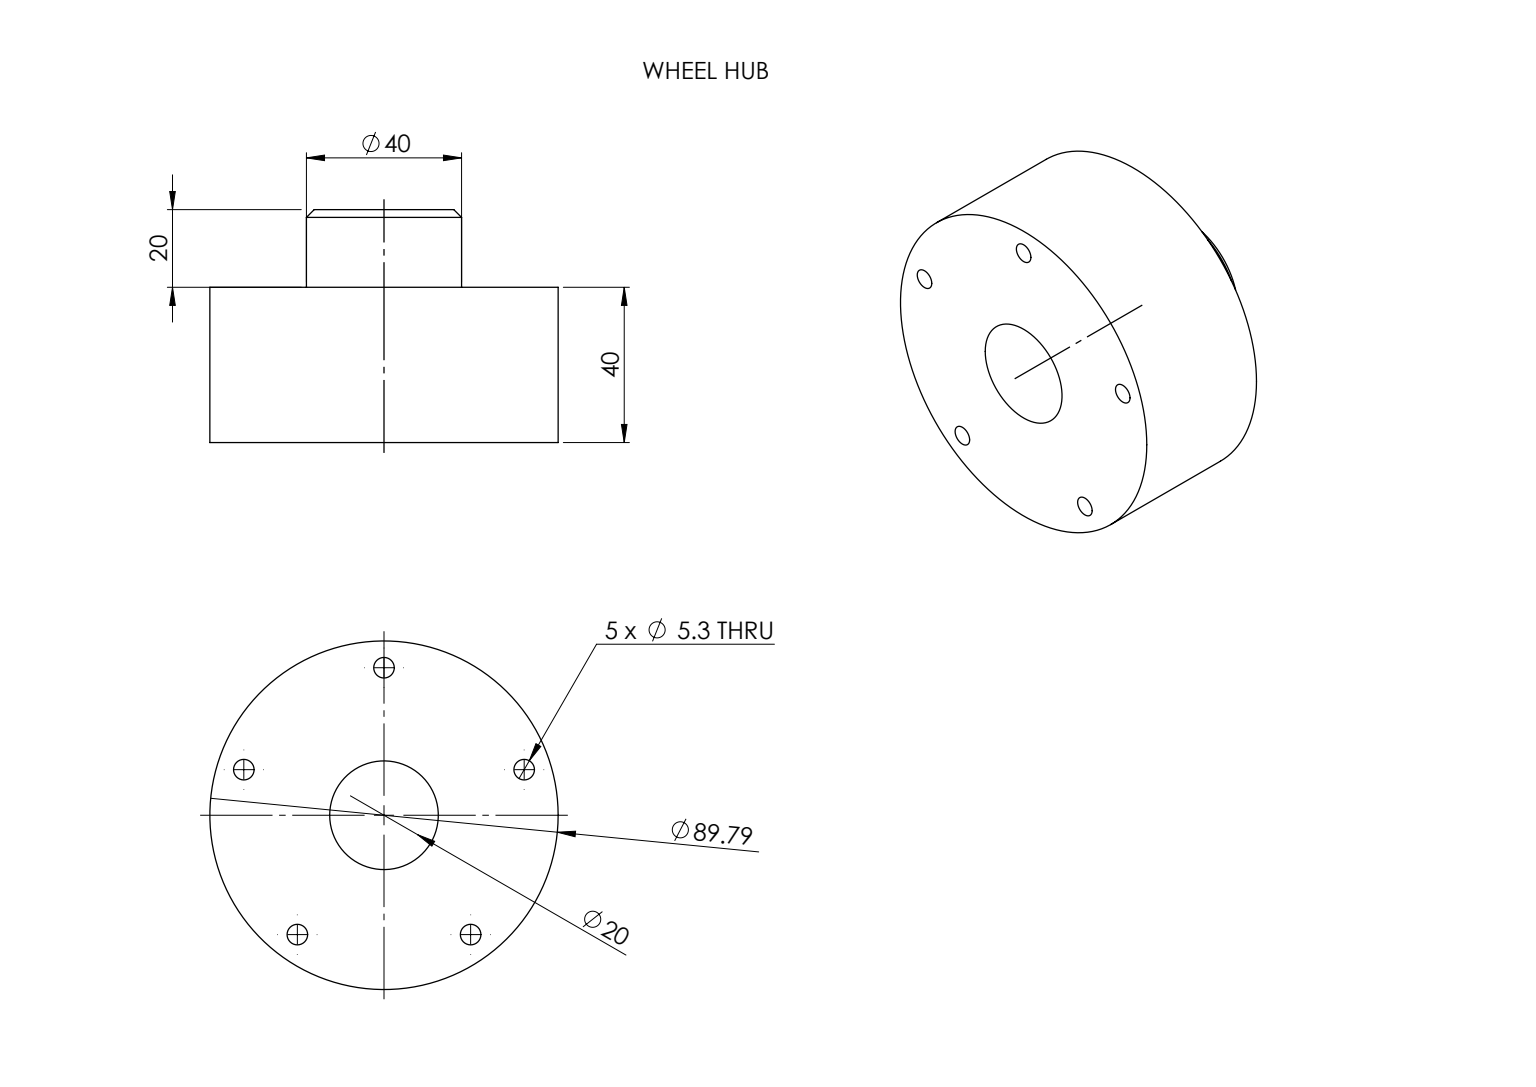
ISO-10303-21;
HEADER;
FILE_DESCRIPTION (('STEP AP214'),
    '1' );
FILE_NAME ('wheel hub.step',
    '2026-10-02T06:35:35',
    ( '' ),
    ( '' ),
    'SwSTEP 2.0',
    'SolidWorks 2026',
    '' );
FILE_SCHEMA (( 'AUTOMOTIVE_DESIGN' ));
ENDSEC;

DATA;
#28=CARTESIAN_POINT ( 'NONE',  ( 0.000000000000000000, 0.000000000000000000, -43.49999999999998579 ) ) ;
#49=CARTESIAN_POINT ( 'NONE',  ( 36.14014761921570340, 11.74264578624841171, -25.50000000000000355 ) ) ;
#103=DIRECTION ( 'NONE',  ( -1.000000000000000000, 0.000000000000000000, 0.000000000000000000 ) ) ;
#141=DIRECTION ( 'NONE',  ( -0.000000000000000000, -0.000000000000000000, -1.000000000000000000 ) ) ;
#154=CIRCLE ( 'NONE', #13005, 2.649999999999985700 ) ;
#173=FACE_OUTER_BOUND ( 'NONE', #9202, .T. ) ;
#234=EDGE_LOOP ( 'NONE', ( #1184, #579, #7849, #6661 ) ) ;
#254=EDGE_CURVE ( 'NONE', #13058, #12937, #12889, .T. ) ;
#255=DIRECTION ( 'NONE',  ( 0.000000000000000000, 0.000000000000000000, -1.000000000000000000 ) ) ;
#276=AXIS2_PLACEMENT_3D ( 'NONE', #8832, #3149, #952 ) ;
#289=CIRCLE ( 'NONE', #11702, 2.649999999999985700 ) ;
#296=CARTESIAN_POINT ( 'NONE',  ( 0.000000000000000000, 0.000000000000000000, 0.000000000000000000 ) ) ;
#313=CARTESIAN_POINT ( 'NONE',  ( -2.449293598294708880E-16, 38.00000000000000000, -25.50000000000000355 ) ) ;
#316=ORIENTED_EDGE ( 'NONE', *, *, #9761, .T. ) ;
#332=PLANE ( 'NONE',  #4860 ) ;
#344=EDGE_CURVE ( 'NONE', #7966, #6056, #4085, .T. ) ;
#357=ORIENTED_EDGE ( 'NONE', *, *, #7968, .F. ) ;
#360=DIRECTION ( 'NONE',  ( -0.000000000000000000, -0.000000000000000000, -1.000000000000000000 ) ) ;
#391=CYLINDRICAL_SURFACE ( 'NONE', #8713, 2.649999999999989253 ) ;
#398=CYLINDRICAL_SURFACE ( 'NONE', #7576, 44.89637028918153305 ) ;
#434=CLOSED_SHELL ( 'NONE', ( #8197, #11127, #13290, #14509, #14180, #5659, #1628, #1611, #1202, #2862, #9335, #12100, #8859, #6336, #14665, #11456, #8232, #5781, #3982, #14557, #1671 ) ) ;
#444=EDGE_CURVE ( 'NONE', #1981, #12602, #7473, .T. ) ;
#455=DIRECTION ( 'NONE',  ( 0.7071067811865444641, 0.000000000000000000, 0.7071067811865505703 ) ) ;
#463=AXIS2_PLACEMENT_3D ( 'NONE', #9565, #3739, #8433 ) ;
#496=FACE_BOUND ( 'NONE', #15028, .T. ) ;
#544=ORIENTED_EDGE ( 'NONE', *, *, #254, .F. ) ;
#551=ORIENTED_EDGE ( 'NONE', *, *, #11963, .T. ) ;
#552=AXIS2_PLACEMENT_3D ( 'NONE', #4395, #14868, #5594 ) ;
#569=DIRECTION ( 'NONE',  ( -1.000000000000000000, 0.000000000000000000, 0.000000000000000000 ) ) ;
#579=ORIENTED_EDGE ( 'NONE', *, *, #13350, .F. ) ;
#584=CIRCLE ( 'NONE', #9055, 2.649999999999985700 ) ;
#604=VERTEX_POINT ( 'NONE', #4820 ) ;
#615=AXIS2_PLACEMENT_3D ( 'NONE', #10778, #2654, #11932 ) ;
#664=VERTEX_POINT ( 'NONE', #8004 ) ;
#679=ORIENTED_EDGE ( 'NONE', *, *, #5242, .T. ) ;
#693=FACE_BOUND ( 'NONE', #8642, .T. ) ;
#722=EDGE_CURVE ( 'NONE', #1196, #1453, #2766, .T. ) ;
#729=PRODUCT_DEFINITION_FORMATION_WITH_SPECIFIED_SOURCE ( 'ANY', '', #6312, .NOT_KNOWN. ) ;
#786=DIRECTION ( 'NONE',  ( 0.000000000000000000, 0.000000000000000000, 1.000000000000000000 ) ) ;
#792=EDGE_CURVE ( 'NONE', #9114, #5585, #14918, .T. ) ;
#796=STYLED_ITEM ( 'NONE', ( #2153 ), #14006 ) ;
#811=ORIENTED_EDGE ( 'NONE', *, *, #3044, .F. ) ;
#812=ORIENTED_EDGE ( 'NONE', *, *, #10110, .F. ) ;
#908=( LENGTH_UNIT ( ) NAMED_UNIT ( * ) SI_UNIT ( .MILLI., .METRE. ) );
#943=DIRECTION ( 'NONE',  ( -0.000000000000000000, -0.000000000000000000, 1.000000000000000000 ) ) ;
#952=DIRECTION ( 'NONE',  ( 1.000000000000000000, 0.000000000000000000, 0.000000000000000000 ) ) ;
#971=( NAMED_UNIT ( * ) SI_UNIT ( $, .STERADIAN. ) SOLID_ANGLE_UNIT ( ) );
#1022=EDGE_CURVE ( 'NONE', #664, #4760, #1315, .T. ) ;
#1039=ORIENTED_EDGE ( 'NONE', *, *, #344, .F. ) ;
#1140=CARTESIAN_POINT ( 'NONE',  ( -44.89637028918153305, 0.000000000000000000, 14.49999999999999822 ) ) ;
#1181=DIRECTION ( 'NONE',  ( 1.000000000000000000, 0.000000000000000000, 0.000000000000000000 ) ) ;
#1184=ORIENTED_EDGE ( 'NONE', *, *, #9617, .F. ) ;
#1191=DIRECTION ( 'NONE',  ( 1.000000000000000000, 0.000000000000000000, 0.000000000000000000 ) ) ;
#1196=VERTEX_POINT ( 'NONE', #5098 ) ;
#1202=ADVANCED_FACE ( 'NONE', ( #14284 ), #398, .T. ) ;
#1204=ORIENTED_EDGE ( 'NONE', *, *, #10110, .T. ) ;
#1232=SHAPE_REPRESENTATION ( 'wheel hub', ( #5108 ), #3871 ) ;
#1234=ORIENTED_EDGE ( 'NONE', *, *, #1022, .T. ) ;
#1293=DIRECTION ( 'NONE',  ( -1.000000000000000000, 0.000000000000000000, 0.000000000000000000 ) ) ;
#1296=CARTESIAN_POINT ( 'NONE',  ( 0.000000000000000000, 0.000000000000000000, 14.49999999999999822 ) ) ;
#1304=CARTESIAN_POINT ( 'NONE',  ( -24.98583958711379083, -30.74264578624812927, -25.50000000000000355 ) ) ;
#1315=LINE ( 'NONE', #8211, #7602 ) ;
#1321=VECTOR ( 'NONE', #14261, 1000.000000000000000 ) ;
#1329=DIRECTION ( 'NONE',  ( -0.000000000000000000, -0.000000000000000000, 1.000000000000000000 ) ) ;
#1386=FACE_OUTER_BOUND ( 'NONE', #1406, .T. ) ;
#1405=DIRECTION ( 'NONE',  ( 0.000000000000000000, 0.000000000000000000, 1.000000000000000000 ) ) ;
#1406=EDGE_LOOP ( 'NONE', ( #12272, #2635, #12944, #14162 ) ) ;
#1436=ORIENTED_EDGE ( 'NONE', *, *, #4515, .F. ) ;
#1443=ORIENTED_EDGE ( 'NONE', *, *, #6310, .F. ) ;
#1446=CARTESIAN_POINT ( 'NONE',  ( -20.00000000000000000, 2.449293598294706513E-15, -25.50000000000000355 ) ) ;
#1453=VERTEX_POINT ( 'NONE', #10254 ) ;
#1546=ORIENTED_EDGE ( 'NONE', *, *, #11963, .F. ) ;
#1551=CARTESIAN_POINT ( 'NONE',  ( -19.68583958711381854, -30.74264578624812927, -25.50000000000000355 ) ) ;
#1555=CARTESIAN_POINT ( 'NONE',  ( 0.000000000000000000, 0.000000000000000000, 14.49999999999999822 ) ) ;
#1608=EDGE_CURVE ( 'NONE', #7966, #10117, #11074, .T. ) ;
#1611=ADVANCED_FACE ( 'NONE', ( #6491 ), #11304, .T. ) ;
#1622=VERTEX_POINT ( 'NONE', #1955 ) ;
#1628=ADVANCED_FACE ( 'NONE', ( #10146 ), #6571, .F. ) ;
#1643=CARTESIAN_POINT ( 'NONE',  ( 36.14014761921570340, 11.74264578624841171, 14.49999999999999822 ) ) ;
#1649=DIRECTION ( 'NONE',  ( -1.000000000000000000, 0.000000000000000000, 0.000000000000000000 ) ) ;
#1671=ADVANCED_FACE ( 'NONE', ( #9378 ), #2394, .F. ) ;
#1676=CARTESIAN_POINT ( 'NONE',  ( -2.649999999999989697, 38.00000000000000000, 14.49999999999999822 ) ) ;
#1682=CARTESIAN_POINT ( 'NONE',  ( 0.000000000000000000, 0.000000000000000000, 14.49999999999999822 ) ) ;
#1690=LINE ( 'NONE', #10643, #5808 ) ;
#1691=DIRECTION ( 'NONE',  ( -0.000000000000000000, -0.000000000000000000, -1.000000000000000000 ) ) ;
#1700=UNCERTAINTY_MEASURE_WITH_UNIT (LENGTH_MEASURE( 1.000000000000000082E-05 ), #4612, 'distance_accuracy_value', 'NONE');
#1710=ORIENTED_EDGE ( 'NONE', *, *, #11180, .F. ) ;
#1717=DIRECTION ( 'NONE',  ( 0.000000000000000000, 0.000000000000000000, 1.000000000000000000 ) ) ;
#1726=EDGE_LOOP ( 'NONE', ( #1204, #13812 ) ) ;
#1730=EDGE_LOOP ( 'NONE', ( #14041, #13678 ) ) ;
#1779=ORIENTED_EDGE ( 'NONE', *, *, #2114, .F. ) ;
#1793=DIRECTION ( 'NONE',  ( -0.000000000000000000, -0.000000000000000000, -1.000000000000000000 ) ) ;
#1806=CARTESIAN_POINT ( 'NONE',  ( -33.49014761921589667, 11.74264578624790190, 14.49999999999999822 ) ) ;
#1824=CARTESIAN_POINT ( 'NONE',  ( 33.49014761921571903, 11.74264578624841171, -25.50000000000000355 ) ) ;
#1832=EDGE_CURVE ( 'NONE', #6056, #10604, #12119, .T. ) ;
#1846=EDGE_CURVE ( 'NONE', #7769, #13374, #8379, .T. ) ;
#1850=ORIENTED_EDGE ( 'NONE', *, *, #10596, .T. ) ;
#1877=CARTESIAN_POINT ( 'NONE',  ( 0.000000000000000000, 0.000000000000000000, -25.50000000000000355 ) ) ;
#1880=ORIENTED_EDGE ( 'NONE', *, *, #4327, .F. ) ;
#1893=AXIS2_PLACEMENT_3D ( 'NONE', #9669, #14480, #14253 ) ;
#1901=ORIENTED_EDGE ( 'NONE', *, *, #12563, .F. ) ;
#1915=FACE_OUTER_BOUND ( 'NONE', #7710, .T. ) ;
#1923=AXIS2_PLACEMENT_3D ( 'NONE', #5073, #9687, #2647 ) ;
#1925=CARTESIAN_POINT ( 'NONE',  ( 2.649999999999988809, 38.00000000000000000, 14.49999999999999822 ) ) ;
#1955=CARTESIAN_POINT ( 'NONE',  ( 18.00000000000000355, 0.000000000000000000, -45.50000000000000000 ) ) ;
#1981=VERTEX_POINT ( 'NONE', #11293 ) ;
#1989=ORIENTED_EDGE ( 'NONE', *, *, #11600, .T. ) ;
#2030=DIRECTION ( 'NONE',  ( 0.000000000000000000, 0.000000000000000000, -1.000000000000000000 ) ) ;
#2086=DIRECTION ( 'NONE',  ( 0.000000000000000000, 0.000000000000000000, 1.000000000000000000 ) ) ;
#2106=DIRECTION ( 'NONE',  ( -1.000000000000000000, 0.000000000000000000, 0.000000000000000000 ) ) ;
#2114=EDGE_CURVE ( 'NONE', #1981, #7885, #154, .T. ) ;
#2128=FACE_BOUND ( 'NONE', #5019, .T. ) ;
#2153=PRESENTATION_STYLE_ASSIGNMENT (( #6769 ) ) ;
#2177=EDGE_LOOP ( 'NONE', ( #8294, #8233 ) ) ;
#2191=EDGE_LOOP ( 'NONE', ( #4825, #12319 ) ) ;
#2204=CARTESIAN_POINT ( 'NONE',  ( -22.33583958711380646, -30.74264578624812927, -25.50000000000000355 ) ) ;
#2209=ORIENTED_EDGE ( 'NONE', *, *, #4162, .T. ) ;
#2214=ADVANCED_BREP_SHAPE_REPRESENTATION ( '', ( #14006, #5108 ), #3871 ) ;
#2241=( GEOMETRIC_REPRESENTATION_CONTEXT ( 3 ) GLOBAL_UNCERTAINTY_ASSIGNED_CONTEXT ( ( #10015 ) ) GLOBAL_UNIT_ASSIGNED_CONTEXT ( ( #7698, #14926, #4667 ) ) REPRESENTATION_CONTEXT ( 'NONE', 'WORKASPACE' ) );
#2250=ORIENTED_EDGE ( 'NONE', *, *, #3584, .T. ) ;
#2269=AXIS2_PLACEMENT_3D ( 'NONE', #6255, #9750, #1649 ) ;
#2276=CIRCLE ( 'NONE', #5174, 20.00000000000000000 ) ;
#2345=LINE ( 'NONE', #8039, #3777 ) ;
#2394=CYLINDRICAL_SURFACE ( 'NONE', #7407, 2.649999999999985700 ) ;
#2405=STYLED_ITEM ( 'NONE', ( #4687 ), #2214 ) ;
#2415=CARTESIAN_POINT ( 'NONE',  ( 36.14014761921570340, 11.74264578624841171, -25.50000000000000355 ) ) ;
#2459=CIRCLE ( 'NONE', #276, 44.89637028918153305 ) ;
#2463=ORIENTED_EDGE ( 'NONE', *, *, #4676, .T. ) ;
#2491=CARTESIAN_POINT ( 'NONE',  ( -22.33583958711380646, -30.74264578624812927, -25.50000000000000355 ) ) ;
#2492=CARTESIAN_POINT ( 'NONE',  ( 44.89637028918153305, 5.498219616798048790E-15, -25.50000000000000355 ) ) ;
#2553=CONICAL_SURFACE ( 'NONE', #13470, 18.00000000000000355, 0.7853981633974439491 ) ;
#2572=CARTESIAN_POINT ( 'NONE',  ( 38.79014761921568777, 11.74264578624841171, -25.50000000000000355 ) ) ;
#2635=ORIENTED_EDGE ( 'NONE', *, *, #3584, .F. ) ;
#2647=DIRECTION ( 'NONE',  ( -1.000000000000000000, 0.000000000000000000, 0.000000000000000000 ) ) ;
#2654=DIRECTION ( 'NONE',  ( 0.000000000000000000, 0.000000000000000000, -1.000000000000000000 ) ) ;
#2674=CYLINDRICAL_SURFACE ( 'NONE', #13644, 2.649999999999985700 ) ;
#2675=CIRCLE ( 'NONE', #4388, 18.00000000000000355 ) ;
#2689=CIRCLE ( 'NONE', #6303, 14.00000000000000000 ) ;
#2708=ORIENTED_EDGE ( 'NONE', *, *, #6734, .F. ) ;
#2727=CIRCLE ( 'NONE', #13165, 2.649999999999985700 ) ;
#2741=DIRECTION ( 'NONE',  ( 0.000000000000000000, 0.000000000000000000, 1.000000000000000000 ) ) ;
#2753=DIRECTION ( 'NONE',  ( 1.000000000000000000, 0.000000000000000000, 0.000000000000000000 ) ) ;
#2764=VERTEX_POINT ( 'NONE', #2970 ) ;
#2766=LINE ( 'NONE', #5196, #7374 ) ;
#2770=CIRCLE ( 'NONE', #11262, 20.00000000000000000 ) ;
#2861=EDGE_CURVE ( 'NONE', #14730, #11825, #5168, .T. ) ;
#2862=ADVANCED_FACE ( 'NONE', ( #8807 ), #5401, .T. ) ;
#2883=DIRECTION ( 'NONE',  ( 1.000000000000000000, 0.000000000000000000, 0.000000000000000000 ) ) ;
#2888=CIRCLE ( 'NONE', #11630, 2.649999999999985700 ) ;
#2911=DIRECTION ( 'NONE',  ( -0.7071067811865444641, 8.659560562354895880E-17, 0.7071067811865505703 ) ) ;
#2926=CARTESIAN_POINT ( 'NONE',  ( -2.449293598294708880E-16, 38.00000000000000000, -25.50000000000000355 ) ) ;
#2939=AXIS2_PLACEMENT_3D ( 'NONE', #10520, #13958, #9300 ) ;
#2954=ORIENTED_EDGE ( 'NONE', *, *, #3044, .T. ) ;
#2970=CARTESIAN_POINT ( 'NONE',  ( 24.98583958711423492, -30.74264578624780597, -25.50000000000000355 ) ) ;
#2993=EDGE_CURVE ( 'NONE', #5519, #12602, #14641, .T. ) ;
#3006=EDGE_LOOP ( 'NONE', ( #12500, #11613, #5941, #2708 ) ) ;
#3033=DIRECTION ( 'NONE',  ( -0.000000000000000000, -0.000000000000000000, -1.000000000000000000 ) ) ;
#3044=EDGE_CURVE ( 'NONE', #2764, #4760, #10509, .T. ) ;
#3054=DIRECTION ( 'NONE',  ( -0.000000000000000000, -0.000000000000000000, -1.000000000000000000 ) ) ;
#3093=EDGE_LOOP ( 'NONE', ( #8891, #811 ) ) ;
#3136=CIRCLE ( 'NONE', #463, 2.649999999999985700 ) ;
#3149=DIRECTION ( 'NONE',  ( 0.000000000000000000, 0.000000000000000000, 1.000000000000000000 ) ) ;
#3265=CARTESIAN_POINT ( 'NONE',  ( 20.00000000000000000, 0.000000000000000000, -43.49999999999998579 ) ) ;
#3286=FACE_OUTER_BOUND ( 'NONE', #11438, .T. ) ;
#3290=CARTESIAN_POINT ( 'NONE',  ( -44.89637028918153305, 0.000000000000000000, -25.50000000000000355 ) ) ;
#3343=FACE_OUTER_BOUND ( 'NONE', #2177, .T. ) ;
#3358=CARTESIAN_POINT ( 'NONE',  ( 0.000000000000000000, 0.000000000000000000, -45.50000000000000000 ) ) ;
#3423=AXIS2_PLACEMENT_3D ( 'NONE', #3994, #10968, #569 ) ;
#3454=DIRECTION ( 'NONE',  ( -1.000000000000000000, 0.000000000000000000, 0.000000000000000000 ) ) ;
#3484=ORIENTED_EDGE ( 'NONE', *, *, #11180, .T. ) ;
#3493=CIRCLE ( 'NONE', #14885, 2.649999999999987477 ) ;
#3511=DIRECTION ( 'NONE',  ( -0.000000000000000000, -0.000000000000000000, -1.000000000000000000 ) ) ;
#3547=AXIS2_PLACEMENT_3D ( 'NONE', #8936, #13571, #12674 ) ;
#3584=EDGE_CURVE ( 'NONE', #604, #11699, #8061, .T. ) ;
#3670=DIRECTION ( 'NONE',  ( -0.000000000000000000, -0.000000000000000000, -1.000000000000000000 ) ) ;
#3688=DIRECTION ( 'NONE',  ( 0.000000000000000000, 0.000000000000000000, -1.000000000000000000 ) ) ;
#3693=ORIENTED_EDGE ( 'NONE', *, *, #10596, .F. ) ;
#3722=AXIS2_PLACEMENT_3D ( 'NONE', #15014, #7091, #1191 ) ;
#3728=AXIS2_PLACEMENT_3D ( 'NONE', #13448, #7669, #12314 ) ;
#3739=DIRECTION ( 'NONE',  ( -0.000000000000000000, -0.000000000000000000, -1.000000000000000000 ) ) ;
#3746=DIRECTION ( 'NONE',  ( -1.000000000000000000, 0.000000000000000000, 0.000000000000000000 ) ) ;
#3748=LINE ( 'NONE', #7370, #9772 ) ;
#3777=VECTOR ( 'NONE', #12681, 1000.000000000000000 ) ;
#3779=FACE_BOUND ( 'NONE', #8908, .T. ) ;
#3783=ORIENTED_EDGE ( 'NONE', *, *, #9761, .F. ) ;
#3787=CARTESIAN_POINT ( 'NONE',  ( -14.00000000000000000, 0.000000000000000000, -45.50000000000000000 ) ) ;
#3850=PRODUCT_DEFINITION ( 'UNKNOWN', '', #729, #11088 ) ;
#3871=( GEOMETRIC_REPRESENTATION_CONTEXT ( 3 ) GLOBAL_UNCERTAINTY_ASSIGNED_CONTEXT ( ( #13249 ) ) GLOBAL_UNIT_ASSIGNED_CONTEXT ( ( #908, #6949, #971 ) ) REPRESENTATION_CONTEXT ( 'NONE', 'WORKASPACE' ) );
#3878=DIRECTION ( 'NONE',  ( -1.000000000000000000, 0.000000000000000000, 0.000000000000000000 ) ) ;
#3905=DIRECTION ( 'NONE',  ( -1.000000000000000000, 0.000000000000000000, 0.000000000000000000 ) ) ;
#3907=DIRECTION ( 'NONE',  ( -1.000000000000000000, 0.000000000000000000, 0.000000000000000000 ) ) ;
#3929=EDGE_LOOP ( 'NONE', ( #14003, #12873, #4799, #14019 ) ) ;
#3977=CARTESIAN_POINT ( 'NONE',  ( 22.33583958711425055, -30.74264578624780597, -25.50000000000000355 ) ) ;
#3982=ADVANCED_FACE ( 'NONE', ( #173 ), #2674, .F. ) ;
#3992=ORIENTED_EDGE ( 'NONE', *, *, #4162, .F. ) ;
#3994=CARTESIAN_POINT ( 'NONE',  ( -36.14014761921588104, 11.74264578624790190, -25.50000000000000355 ) ) ;
#3996=CARTESIAN_POINT ( 'NONE',  ( -38.79014761921587251, 11.74264578624790190, 14.49999999999999822 ) ) ;
#4044=DIRECTION ( 'NONE',  ( -0.000000000000000000, -0.000000000000000000, -1.000000000000000000 ) ) ;
#4066=ORIENTED_EDGE ( 'NONE', *, *, #12665, .F. ) ;
#4078=ORIENTED_EDGE ( 'NONE', *, *, #8401, .T. ) ;
#4085=CIRCLE ( 'NONE', #1893, 2.649999999999989253 ) ;
#4162=EDGE_CURVE ( 'NONE', #5875, #10752, #6907, .T. ) ;
#4173=DIRECTION ( 'NONE',  ( -0.000000000000000000, -0.000000000000000000, -1.000000000000000000 ) ) ;
#4193=FACE_BOUND ( 'NONE', #8365, .T. ) ;
#4196=DIRECTION ( 'NONE',  ( -1.000000000000000000, 0.000000000000000000, 0.000000000000000000 ) ) ;
#4203=ORIENTED_EDGE ( 'NONE', *, *, #1608, .F. ) ;
#4208=DIRECTION ( 'NONE',  ( -0.000000000000000000, -0.000000000000000000, 1.000000000000000000 ) ) ;
#4248=CARTESIAN_POINT ( 'NONE',  ( 0.000000000000000000, 0.000000000000000000, -45.50000000000000000 ) ) ;
#4255=AXIS2_PLACEMENT_3D ( 'NONE', #5276, #2086, #9894 ) ;
#4287=CARTESIAN_POINT ( 'NONE',  ( 20.00000000000000000, 0.000000000000000000, -45.50000000000000000 ) ) ;
#4307=ORIENTED_EDGE ( 'NONE', *, *, #7924, .F. ) ;
#4327=EDGE_CURVE ( 'NONE', #5762, #13414, #11773, .T. ) ;
#4388=AXIS2_PLACEMENT_3D ( 'NONE', #6352, #9557, #3878 ) ;
#4394=CARTESIAN_POINT ( 'NONE',  ( 38.79014761921568777, 11.74264578624841171, -25.50000000000000355 ) ) ;
#4395=CARTESIAN_POINT ( 'NONE',  ( 0.000000000000000000, 0.000000000000000000, 14.49999999999999822 ) ) ;
#4424=ORIENTED_EDGE ( 'NONE', *, *, #2993, .T. ) ;
#4435=DIRECTION ( 'NONE',  ( 1.000000000000000000, 0.000000000000000000, 0.000000000000000000 ) ) ;
#4472=AXIS2_PLACEMENT_3D ( 'NONE', #8660, #8887, #13521 ) ;
#4488=DIRECTION ( 'NONE',  ( 0.000000000000000000, 0.000000000000000000, 1.000000000000000000 ) ) ;
#4503=AXIS2_PLACEMENT_3D ( 'NONE', #5177, #14515, #9791 ) ;
#4512=AXIS2_PLACEMENT_3D ( 'NONE', #1643, #1717, #13263 ) ;
#4515=EDGE_CURVE ( 'NONE', #6851, #13058, #5229, .T. ) ;
#4565=DIRECTION ( 'NONE',  ( 1.000000000000000000, 0.000000000000000000, -0.000000000000000000 ) ) ;
#4575=DIRECTION ( 'NONE',  ( -1.000000000000000000, 0.000000000000000000, 0.000000000000000000 ) ) ;
#4586=VERTEX_POINT ( 'NONE', #13813 ) ;
#4612=( LENGTH_UNIT ( ) NAMED_UNIT ( * ) SI_UNIT ( .MILLI., .METRE. ) );
#4615=AXIS2_PLACEMENT_3D ( 'NONE', #13859, #10426, #3454 ) ;
#4617=DIRECTION ( 'NONE',  ( -0.000000000000000000, -0.000000000000000000, -1.000000000000000000 ) ) ;
#4632=AXIS2_PLACEMENT_3D ( 'NONE', #1296, #7042, #4565 ) ;
#4645=CIRCLE ( 'NONE', #9712, 2.649999999999985700 ) ;
#4667=( NAMED_UNIT ( * ) SI_UNIT ( $, .STERADIAN. ) SOLID_ANGLE_UNIT ( ) );
#4676=EDGE_CURVE ( 'NONE', #11699, #13414, #9535, .T. ) ;
#4687=PRESENTATION_STYLE_ASSIGNMENT (( #14788 ) ) ;
#4760=VERTEX_POINT ( 'NONE', #7103 ) ;
#4784=FACE_OUTER_BOUND ( 'NONE', #11618, .T. ) ;
#4796=CARTESIAN_POINT ( 'NONE',  ( 33.49014761921571903, 11.74264578624841171, 14.49999999999999822 ) ) ;
#4799=ORIENTED_EDGE ( 'NONE', *, *, #11826, .T. ) ;
#4804=VECTOR ( 'NONE', #5750, 1000.000000000000000 ) ;
#4820=CARTESIAN_POINT ( 'NONE',  ( -14.00000000000000000, 0.000000000000000000, 14.49999999999999822 ) ) ;
#4825=ORIENTED_EDGE ( 'NONE', *, *, #7977, .F. ) ;
#4834=DIRECTION ( 'NONE',  ( -0.000000000000000000, -0.000000000000000000, -1.000000000000000000 ) ) ;
#4860=AXIS2_PLACEMENT_3D ( 'NONE', #10728, #6164, #13241 ) ;
#4871=CYLINDRICAL_SURFACE ( 'NONE', #6660, 2.649999999999989253 ) ;
#4970=FACE_BOUND ( 'NONE', #5840, .T. ) ;
#5006=EDGE_LOOP ( 'NONE', ( #6244, #9510, #13738, #4424 ) ) ;
#5019=EDGE_LOOP ( 'NONE', ( #1039, #1546 ) ) ;
#5044=CARTESIAN_POINT ( 'NONE',  ( 0.000000000000000000, 0.000000000000000000, -25.50000000000000355 ) ) ;
#5073=CARTESIAN_POINT ( 'NONE',  ( 0.000000000000000000, 0.000000000000000000, 14.49999999999999822 ) ) ;
#5095=AXIS2_PLACEMENT_3D ( 'NONE', #14277, #7434, #7357 ) ;
#5098=CARTESIAN_POINT ( 'NONE',  ( -18.00000000000000355, 2.326828918379971365E-15, -45.50000000000000000 ) ) ;
#5108=AXIS2_PLACEMENT_3D ( 'NONE', #296, #6125, #10768 ) ;
#5168=CIRCLE ( 'NONE', #6618, 2.649999999999985700 ) ;
#5174=AXIS2_PLACEMENT_3D ( 'NONE', #12943, #1405, #6092 ) ;
#5177=CARTESIAN_POINT ( 'NONE',  ( -36.14014761921588104, 11.74264578624790190, 14.49999999999999822 ) ) ;
#5196=CARTESIAN_POINT ( 'NONE',  ( -18.00000000000000355, 2.204364238465235822E-15, -45.50000000000000000 ) ) ;
#5205=LINE ( 'NONE', #8259, #10473 ) ;
#5229=CIRCLE ( 'NONE', #3547, 44.89637028918153305 ) ;
#5236=APPLICATION_CONTEXT ( 'automotive_design' ) ;
#5242=EDGE_CURVE ( 'NONE', #7769, #14730, #3748, .T. ) ;
#5276=CARTESIAN_POINT ( 'NONE',  ( 0.000000000000000000, 0.000000000000000000, -25.50000000000000355 ) ) ;
#5296=CARTESIAN_POINT ( 'NONE',  ( -2.649999999999989697, 38.00000000000000000, -25.50000000000000355 ) ) ;
#5324=ORIENTED_EDGE ( 'NONE', *, *, #11600, .F. ) ;
#5333=CIRCLE ( 'NONE', #4615, 2.649999999999985700 ) ;
#5334=CARTESIAN_POINT ( 'NONE',  ( -38.79014761921587251, 11.74264578624790190, -25.50000000000000355 ) ) ;
#5338=CYLINDRICAL_SURFACE ( 'NONE', #13383, 20.00000000000000000 ) ;
#5348=ORIENTED_EDGE ( 'NONE', *, *, #14320, .T. ) ;
#5367=EDGE_CURVE ( 'NONE', #12937, #11617, #11006, .T. ) ;
#5386=CARTESIAN_POINT ( 'NONE',  ( 44.89637028918153305, 5.498219616798048790E-15, 14.49999999999999822 ) ) ;
#5401=CYLINDRICAL_SURFACE ( 'NONE', #3728, 44.89637028918153305 ) ;
#5481=EDGE_LOOP ( 'NONE', ( #1436, #10869, #10187, #544 ) ) ;
#5519=VERTEX_POINT ( 'NONE', #8425 ) ;
#5526=DIRECTION ( 'NONE',  ( 1.000000000000000000, 0.000000000000000000, 0.000000000000000000 ) ) ;
#5562=EDGE_LOOP ( 'NONE', ( #9322, #316, #679, #9636 ) ) ;
#5580=CARTESIAN_POINT ( 'NONE',  ( -22.33583958711380646, -30.74264578624812927, 14.49999999999999822 ) ) ;
#5585=VERTEX_POINT ( 'NONE', #1446 ) ;
#5594=DIRECTION ( 'NONE',  ( -1.000000000000000000, 0.000000000000000000, 0.000000000000000000 ) ) ;
#5649=DIRECTION ( 'NONE',  ( 0.000000000000000000, 0.000000000000000000, 1.000000000000000000 ) ) ;
#5659=ADVANCED_FACE ( 'NONE', ( #6802 ), #11754, .T. ) ;
#5676=CARTESIAN_POINT ( 'NONE',  ( 0.000000000000000000, 0.000000000000000000, -45.50000000000000000 ) ) ;
#5744=DIRECTION ( 'NONE',  ( -0.000000000000000000, -0.000000000000000000, -1.000000000000000000 ) ) ;
#5750=DIRECTION ( 'NONE',  ( -0.000000000000000000, -0.000000000000000000, -1.000000000000000000 ) ) ;
#5762=VERTEX_POINT ( 'NONE', #3787 ) ;
#5781=ADVANCED_FACE ( 'NONE', ( #14318 ), #12057, .F. ) ;
#5805=SHAPE_REPRESENTATION_RELATIONSHIP ( 'NONE' , 'NONE' ,  #1232, #2214 ) ;
#5808=VECTOR ( 'NONE', #7448, 1000.000000000000000 ) ;
#5809=CARTESIAN_POINT ( 'NONE',  ( -2.449293598294708880E-16, 38.00000000000000000, -25.50000000000000355 ) ) ;
#5840=EDGE_LOOP ( 'NONE', ( #1880, #3693 ) ) ;
#5875=VERTEX_POINT ( 'NONE', #3996 ) ;
#5922=DIRECTION ( 'NONE',  ( -0.000000000000000000, -0.000000000000000000, -1.000000000000000000 ) ) ;
#5941=ORIENTED_EDGE ( 'NONE', *, *, #6210, .F. ) ;
#5957=CARTESIAN_POINT ( 'NONE',  ( 0.000000000000000000, 0.000000000000000000, -25.50000000000000355 ) ) ;
#5980=CARTESIAN_POINT ( 'NONE',  ( 22.33583958711425055, -30.74264578624780597, 14.49999999999999822 ) ) ;
#5982=ORIENTED_EDGE ( 'NONE', *, *, #7977, .T. ) ;
#6012=EDGE_CURVE ( 'NONE', #11617, #12937, #8599, .T. ) ;
#6025=FACE_BOUND ( 'NONE', #3093, .T. ) ;
#6045=LINE ( 'NONE', #2572, #1321 ) ;
#6056=VERTEX_POINT ( 'NONE', #1925 ) ;
#6085=APPLICATION_CONTEXT ( 'automotive_design' ) ;
#6092=DIRECTION ( 'NONE',  ( -1.000000000000000000, 0.000000000000000000, 0.000000000000000000 ) ) ;
#6101=ORIENTED_EDGE ( 'NONE', *, *, #6734, .T. ) ;
#6117=CARTESIAN_POINT ( 'NONE',  ( -19.68583958711381854, -30.74264578624812927, -25.50000000000000355 ) ) ;
#6125=DIRECTION ( 'NONE',  ( 0.000000000000000000, 0.000000000000000000, 1.000000000000000000 ) ) ;
#6158=EDGE_LOOP ( 'NONE', ( #8298, #9643, #7961, #4203 ) ) ;
#6164=DIRECTION ( 'NONE',  ( 0.000000000000000000, 0.000000000000000000, -1.000000000000000000 ) ) ;
#6167=CARTESIAN_POINT ( 'NONE',  ( -20.00000000000000000, 2.449293598294706513E-15, -45.50000000000000000 ) ) ;
#6174=VECTOR ( 'NONE', #6977, 1000.000000000000000 ) ;
#6201=CARTESIAN_POINT ( 'NONE',  ( 14.00000000000000000, 1.714505518806294638E-15, 14.49999999999999822 ) ) ;
#6210=EDGE_CURVE ( 'NONE', #11466, #1453, #11158, .T. ) ;
#6215=LINE ( 'NONE', #14276, #9954 ) ;
#6230=EDGE_CURVE ( 'NONE', #4760, #2764, #5333, .T. ) ;
#6244=ORIENTED_EDGE ( 'NONE', *, *, #444, .F. ) ;
#6252=ORIENTED_EDGE ( 'NONE', *, *, #7073, .T. ) ;
#6255=CARTESIAN_POINT ( 'NONE',  ( 22.33583958711425055, -30.74264578624780597, -25.50000000000000355 ) ) ;
#6303=AXIS2_PLACEMENT_3D ( 'NONE', #11839, #8553, #11919 ) ;
#6310=EDGE_CURVE ( 'NONE', #604, #5762, #1690, .T. ) ;
#6312=PRODUCT ( 'wheel hub', 'wheel hub', '', ( #9272 ) ) ;
#6316=CIRCLE ( 'NONE', #7047, 2.649999999999987477 ) ;
#6336=ADVANCED_FACE ( 'NONE', ( #8590, #4970 ), #332, .T. ) ;
#6352=CARTESIAN_POINT ( 'NONE',  ( 0.000000000000000000, 0.000000000000000000, -45.50000000000000000 ) ) ;
#6398=ORIENTED_EDGE ( 'NONE', *, *, #8604, .F. ) ;
#6401=DIRECTION ( 'NONE',  ( -1.000000000000000000, 0.000000000000000000, 0.000000000000000000 ) ) ;
#6441=EDGE_LOOP ( 'NONE', ( #13074, #11099 ) ) ;
#6491=FACE_OUTER_BOUND ( 'NONE', #3929, .T. ) ;
#6506=FACE_OUTER_BOUND ( 'NONE', #9509, .T. ) ;
#6571=CYLINDRICAL_SURFACE ( 'NONE', #552, 14.00000000000000000 ) ;
#6618=AXIS2_PLACEMENT_3D ( 'NONE', #14596, #3054, #4196 ) ;
#6623=CIRCLE ( 'NONE', #12454, 18.00000000000000355 ) ;
#6660=AXIS2_PLACEMENT_3D ( 'NONE', #9188, #5922, #8357 ) ;
#6661=ORIENTED_EDGE ( 'NONE', *, *, #5367, .T. ) ;
#6667=DIRECTION ( 'NONE',  ( 1.000000000000000000, 0.000000000000000000, 0.000000000000000000 ) ) ;
#6716=ORIENTED_EDGE ( 'NONE', *, *, #8401, .F. ) ;
#6734=EDGE_CURVE ( 'NONE', #1622, #11466, #6215, .T. ) ;
#6737=DIRECTION ( 'NONE',  ( -0.000000000000000000, -0.000000000000000000, -1.000000000000000000 ) ) ;
#6769=SURFACE_STYLE_USAGE ( .BOTH. , #7925 ) ;
#6793=SURFACE_STYLE_FILL_AREA ( #12740 ) ;
#6802=FACE_OUTER_BOUND ( 'NONE', #3006, .T. ) ;
#6816=CARTESIAN_POINT ( 'NONE',  ( 22.33583958711425055, -30.74264578624780597, -25.50000000000000355 ) ) ;
#6820=DIRECTION ( 'NONE',  ( -0.000000000000000000, -0.000000000000000000, -1.000000000000000000 ) ) ;
#6851=VERTEX_POINT ( 'NONE', #8018 ) ;
#6877=DIRECTION ( 'NONE',  ( -1.000000000000000000, 0.000000000000000000, 0.000000000000000000 ) ) ;
#6896=CYLINDRICAL_SURFACE ( 'NONE', #13564, 2.649999999999985700 ) ;
#6907=CIRCLE ( 'NONE', #4503, 2.649999999999985700 ) ;
#6949=( NAMED_UNIT ( * ) PLANE_ANGLE_UNIT ( ) SI_UNIT ( $, .RADIAN. ) );
#6977=DIRECTION ( 'NONE',  ( -0.000000000000000000, -0.000000000000000000, -1.000000000000000000 ) ) ;
#7015=AXIS2_PLACEMENT_3D ( 'NONE', #28, #5649, #103 ) ;
#7042=DIRECTION ( 'NONE',  ( 0.000000000000000000, 0.000000000000000000, 1.000000000000000000 ) ) ;
#7047=AXIS2_PLACEMENT_3D ( 'NONE', #5809, #12811, #11542 ) ;
#7054=CYLINDRICAL_SURFACE ( 'NONE', #10657, 2.649999999999985700 ) ;
#7073=EDGE_CURVE ( 'NONE', #10743, #7688, #7293, .T. ) ;
#7083=ORIENTED_EDGE ( 'NONE', *, *, #444, .T. ) ;
#7091=DIRECTION ( 'NONE',  ( 0.000000000000000000, 0.000000000000000000, 1.000000000000000000 ) ) ;
#7103=CARTESIAN_POINT ( 'NONE',  ( 19.68583958711426263, -30.74264578624780597, -25.50000000000000355 ) ) ;
#7153=VECTOR ( 'NONE', #7321, 1000.000000000000000 ) ;
#7172=CARTESIAN_POINT ( 'NONE',  ( 2.649999999999988809, 38.00000000000000000, -25.50000000000000355 ) ) ;
#7207=FACE_OUTER_BOUND ( 'NONE', #12076, .T. ) ;
#7216=DIRECTION ( 'NONE',  ( -1.000000000000000000, 0.000000000000000000, 0.000000000000000000 ) ) ;
#7232=CIRCLE ( 'NONE', #10403, 2.649999999999985700 ) ;
#7293=CIRCLE ( 'NONE', #2939, 2.649999999999985700 ) ;
#7300=CYLINDRICAL_SURFACE ( 'NONE', #10970, 2.649999999999985700 ) ;
#7307=COLOUR_RGB ( '', 0.08235294, 0.09019608, 0.10196078) ;
#7320=DIRECTION ( 'NONE',  ( 1.000000000000000000, 0.000000000000000000, -0.000000000000000000 ) ) ;
#7321=DIRECTION ( 'NONE',  ( -0.000000000000000000, -0.000000000000000000, -1.000000000000000000 ) ) ;
#7327=CARTESIAN_POINT ( 'NONE',  ( -22.33583958711380646, -30.74264578624812927, -25.50000000000000355 ) ) ;
#7357=DIRECTION ( 'NONE',  ( -1.000000000000000000, 0.000000000000000000, 0.000000000000000000 ) ) ;
#7370=CARTESIAN_POINT ( 'NONE',  ( 33.49014761921571903, 11.74264578624841171, -25.50000000000000355 ) ) ;
#7372=VECTOR ( 'NONE', #360, 1000.000000000000000 ) ;
#7374=VECTOR ( 'NONE', #2911, 1000.000000000000000 ) ;
#7379=FACE_OUTER_BOUND ( 'NONE', #11819, .T. ) ;
#7407=AXIS2_PLACEMENT_3D ( 'NONE', #49, #5744, #8021 ) ;
#7434=DIRECTION ( 'NONE',  ( -0.000000000000000000, -0.000000000000000000, -1.000000000000000000 ) ) ;
#7448=DIRECTION ( 'NONE',  ( -0.000000000000000000, -0.000000000000000000, -1.000000000000000000 ) ) ;
#7473=LINE ( 'NONE', #6117, #7372 ) ;
#7478=ORIENTED_EDGE ( 'NONE', *, *, #14359, .T. ) ;
#7533=PRODUCT_DEFINITION_SHAPE ( 'NONE', 'NONE',  #3850 ) ;
#7576=AXIS2_PLACEMENT_3D ( 'NONE', #1682, #4044, #3746 ) ;
#7596=ORIENTED_EDGE ( 'NONE', *, *, #11684, .T. ) ;
#7602=VECTOR ( 'NONE', #12927, 1000.000000000000000 ) ;
#7629=AXIS2_PLACEMENT_3D ( 'NONE', #7327, #4834, #14398 ) ;
#7659=ORIENTED_EDGE ( 'NONE', *, *, #14359, .F. ) ;
#7669=DIRECTION ( 'NONE',  ( -0.000000000000000000, -0.000000000000000000, -1.000000000000000000 ) ) ;
#7688=VERTEX_POINT ( 'NONE', #5334 ) ;
#7698=( LENGTH_UNIT ( ) NAMED_UNIT ( * ) SI_UNIT ( .MILLI., .METRE. ) );
#7710=EDGE_LOOP ( 'NONE', ( #4066, #10920, #5348, #8639 ) ) ;
#7750=DIRECTION ( 'NONE',  ( 1.000000000000000000, 0.000000000000000000, 0.000000000000000000 ) ) ;
#7769=VERTEX_POINT ( 'NONE', #4796 ) ;
#7820=CIRCLE ( 'NONE', #3722, 2.649999999999989253 ) ;
#7849=ORIENTED_EDGE ( 'NONE', *, *, #254, .T. ) ;
#7885=VERTEX_POINT ( 'NONE', #12084 ) ;
#7924=EDGE_CURVE ( 'NONE', #7885, #1981, #7232, .T. ) ;
#7925=SURFACE_SIDE_STYLE ('',( #12274 ) ) ;
#7959=FACE_OUTER_BOUND ( 'NONE', #9307, .T. ) ;
#7961=ORIENTED_EDGE ( 'NONE', *, *, #12347, .T. ) ;
#7966=VERTEX_POINT ( 'NONE', #1676 ) ;
#7968=EDGE_CURVE ( 'NONE', #11825, #14730, #3136, .T. ) ;
#7977=EDGE_CURVE ( 'NONE', #664, #4586, #2888, .T. ) ;
#8004=CARTESIAN_POINT ( 'NONE',  ( 19.68583958711426263, -30.74264578624780597, 14.49999999999999822 ) ) ;
#8018=CARTESIAN_POINT ( 'NONE',  ( 44.89637028918153305, 5.498219616798048790E-15, 14.49999999999999822 ) ) ;
#8021=DIRECTION ( 'NONE',  ( -1.000000000000000000, 0.000000000000000000, 0.000000000000000000 ) ) ;
#8039=CARTESIAN_POINT ( 'NONE',  ( -33.49014761921589667, 11.74264578624790190, -25.50000000000000355 ) ) ;
#8042=CYLINDRICAL_SURFACE ( 'NONE', #9193, 2.649999999999985700 ) ;
#8061=CIRCLE ( 'NONE', #9998, 14.00000000000000000 ) ;
#8197=ADVANCED_FACE ( 'NONE', ( #4784 ), #8042, .F. ) ;
#8202=CARTESIAN_POINT ( 'NONE',  ( 24.98583958711423492, -30.74264578624780597, -25.50000000000000355 ) ) ;
#8211=CARTESIAN_POINT ( 'NONE',  ( 19.68583958711426263, -30.74264578624780597, -25.50000000000000355 ) ) ;
#8232=ADVANCED_FACE ( 'NONE', ( #7959 ), #6896, .F. ) ;
#8233=ORIENTED_EDGE ( 'NONE', *, *, #4515, .T. ) ;
#8259=CARTESIAN_POINT ( 'NONE',  ( -38.79014761921587251, 11.74264578624790190, -25.50000000000000355 ) ) ;
#8294=ORIENTED_EDGE ( 'NONE', *, *, #13350, .T. ) ;
#8298=ORIENTED_EDGE ( 'NONE', *, *, #344, .T. ) ;
#8357=DIRECTION ( 'NONE',  ( -1.000000000000000000, 0.000000000000000000, 0.000000000000000000 ) ) ;
#8362=CARTESIAN_POINT ( 'NONE',  ( 22.33583958711425055, -30.74264578624780597, 14.49999999999999822 ) ) ;
#8364=CARTESIAN_POINT ( 'NONE',  ( 20.00000000000000000, 0.000000000000000000, -25.50000000000000355 ) ) ;
#8365=EDGE_LOOP ( 'NONE', ( #2250, #4078 ) ) ;
#8379=CIRCLE ( 'NONE', #4512, 2.649999999999985700 ) ;
#8397=FACE_BOUND ( 'NONE', #1730, .T. ) ;
#8401=EDGE_CURVE ( 'NONE', #11699, #604, #8467, .T. ) ;
#8425=CARTESIAN_POINT ( 'NONE',  ( -24.98583958711379083, -30.74264578624812927, -25.50000000000000355 ) ) ;
#8433=DIRECTION ( 'NONE',  ( -1.000000000000000000, 0.000000000000000000, 0.000000000000000000 ) ) ;
#8442=ORIENTED_EDGE ( 'NONE', *, *, #1608, .T. ) ;
#8461=FACE_BOUND ( 'NONE', #6441, .T. ) ;
#8467=CIRCLE ( 'NONE', #1923, 14.00000000000000000 ) ;
#8501=DIRECTION ( 'NONE',  ( 0.000000000000000000, 0.000000000000000000, 1.000000000000000000 ) ) ;
#8516=ORIENTED_EDGE ( 'NONE', *, *, #7968, .T. ) ;
#8534=CYLINDRICAL_SURFACE ( 'NONE', #3423, 2.649999999999985700 ) ;
#8553=DIRECTION ( 'NONE',  ( 0.000000000000000000, 0.000000000000000000, -1.000000000000000000 ) ) ;
#8571=DIRECTION ( 'NONE',  ( -0.000000000000000000, -0.000000000000000000, -1.000000000000000000 ) ) ;
#8590=FACE_OUTER_BOUND ( 'NONE', #1726, .T. ) ;
#8599=CIRCLE ( 'NONE', #4255, 44.89637028918153305 ) ;
#8604=EDGE_CURVE ( 'NONE', #10117, #10604, #6316, .T. ) ;
#8625=EDGE_CURVE ( 'NONE', #7688, #10743, #4645, .T. ) ;
#8639=ORIENTED_EDGE ( 'NONE', *, *, #792, .T. ) ;
#8642=EDGE_LOOP ( 'NONE', ( #3992, #7659 ) ) ;
#8660=CARTESIAN_POINT ( 'NONE',  ( 0.000000000000000000, 0.000000000000000000, -25.50000000000000355 ) ) ;
#8705=LINE ( 'NONE', #5386, #11407 ) ;
#8713=AXIS2_PLACEMENT_3D ( 'NONE', #313, #8571, #14213 ) ;
#8807=FACE_OUTER_BOUND ( 'NONE', #234, .T. ) ;
#8832=CARTESIAN_POINT ( 'NONE',  ( 0.000000000000000000, 0.000000000000000000, 14.49999999999999822 ) ) ;
#8836=ORIENTED_EDGE ( 'NONE', *, *, #12347, .F. ) ;
#8859=ADVANCED_FACE ( 'NONE', ( #1915 ), #5338, .T. ) ;
#8887=DIRECTION ( 'NONE',  ( 0.000000000000000000, 0.000000000000000000, 1.000000000000000000 ) ) ;
#8891=ORIENTED_EDGE ( 'NONE', *, *, #6230, .F. ) ;
#8908=EDGE_LOOP ( 'NONE', ( #9874, #14044 ) ) ;
#8936=CARTESIAN_POINT ( 'NONE',  ( 0.000000000000000000, 0.000000000000000000, 14.49999999999999822 ) ) ;
#8950=DIRECTION ( 'NONE',  ( -1.000000000000000000, 0.000000000000000000, 0.000000000000000000 ) ) ;
#8959=AXIS2_PLACEMENT_3D ( 'NONE', #9577, #10726, #2753 ) ;
#9034=AXIS2_PLACEMENT_3D ( 'NONE', #5957, #14312, #7320 ) ;
#9055=AXIS2_PLACEMENT_3D ( 'NONE', #5980, #12904, #11774 ) ;
#9114=VERTEX_POINT ( 'NONE', #8364 ) ;
#9129=ORIENTED_EDGE ( 'NONE', *, *, #13875, .F. ) ;
#9148=DIRECTION ( 'NONE',  ( 0.000000000000000000, 0.000000000000000000, 1.000000000000000000 ) ) ;
#9157=( NAMED_UNIT ( * ) PLANE_ANGLE_UNIT ( ) SI_UNIT ( $, .RADIAN. ) );
#9177=ORIENTED_EDGE ( 'NONE', *, *, #1846, .T. ) ;
#9188=CARTESIAN_POINT ( 'NONE',  ( -2.449293598294708880E-16, 38.00000000000000000, -25.50000000000000355 ) ) ;
#9193=AXIS2_PLACEMENT_3D ( 'NONE', #2415, #6737, #1293 ) ;
#9200=CIRCLE ( 'NONE', #8959, 2.649999999999985700 ) ;
#9202=EDGE_LOOP ( 'NONE', ( #5324, #7478, #9618, #12990 ) ) ;
#9239=DIRECTION ( 'NONE',  ( 1.000000000000000000, 0.000000000000000000, 0.000000000000000000 ) ) ;
#9256=PLANE ( 'NONE',  #4632 ) ;
#9268=LINE ( 'NONE', #8202, #12737 ) ;
#9272=PRODUCT_CONTEXT ( 'NONE', #6085, 'mechanical' ) ;
#9300=DIRECTION ( 'NONE',  ( -1.000000000000000000, 0.000000000000000000, 0.000000000000000000 ) ) ;
#9307=EDGE_LOOP ( 'NONE', ( #1710, #12322, #1234, #12991 ) ) ;
#9322=ORIENTED_EDGE ( 'NONE', *, *, #11684, .F. ) ;
#9324=DIRECTION ( 'NONE',  ( -0.000000000000000000, -0.000000000000000000, -1.000000000000000000 ) ) ;
#9335=ADVANCED_FACE ( 'NONE', ( #12538, #2128, #693, #9942, #14593, #4193, #3343 ), #9256, .T. ) ;
#9378=FACE_OUTER_BOUND ( 'NONE', #5562, .T. ) ;
#9509=EDGE_LOOP ( 'NONE', ( #10769, #812, #6101, #1901 ) ) ;
#9510=ORIENTED_EDGE ( 'NONE', *, *, #2114, .T. ) ;
#9535=LINE ( 'NONE', #11615, #14452 ) ;
#9557=DIRECTION ( 'NONE',  ( 0.000000000000000000, 0.000000000000000000, -1.000000000000000000 ) ) ;
#9565=CARTESIAN_POINT ( 'NONE',  ( 36.14014761921570340, 11.74264578624841171, -25.50000000000000355 ) ) ;
#9577=CARTESIAN_POINT ( 'NONE',  ( 36.14014761921570340, 11.74264578624841171, 14.49999999999999822 ) ) ;
#9617=EDGE_CURVE ( 'NONE', #6851, #11617, #8705, .T. ) ;
#9618=ORIENTED_EDGE ( 'NONE', *, *, #13875, .T. ) ;
#9636=ORIENTED_EDGE ( 'NONE', *, *, #2861, .T. ) ;
#9643=ORIENTED_EDGE ( 'NONE', *, *, #1832, .T. ) ;
#9662=PLANE ( 'NONE',  #9034 ) ;
#9669=CARTESIAN_POINT ( 'NONE',  ( -2.449293598294708880E-16, 38.00000000000000000, 14.49999999999999822 ) ) ;
#9673=ORIENTED_EDGE ( 'NONE', *, *, #6012, .F. ) ;
#9686=CARTESIAN_POINT ( 'NONE',  ( -44.89637028918153305, 0.000000000000000000, 14.49999999999999822 ) ) ;
#9687=DIRECTION ( 'NONE',  ( 0.000000000000000000, 0.000000000000000000, -1.000000000000000000 ) ) ;
#9688=EDGE_LOOP ( 'NONE', ( #11521, #3783 ) ) ;
#9712=AXIS2_PLACEMENT_3D ( 'NONE', #14870, #4617, #6877 ) ;
#9714=CARTESIAN_POINT ( 'NONE',  ( -36.14014761921588104, 11.74264578624790190, -25.50000000000000355 ) ) ;
#9717=DIRECTION ( 'NONE',  ( -0.000000000000000000, -0.000000000000000000, -1.000000000000000000 ) ) ;
#9750=DIRECTION ( 'NONE',  ( -0.000000000000000000, -0.000000000000000000, -1.000000000000000000 ) ) ;
#9761=EDGE_CURVE ( 'NONE', #13374, #7769, #9200, .T. ) ;
#9772=VECTOR ( 'NONE', #9717, 1000.000000000000000 ) ;
#9791=DIRECTION ( 'NONE',  ( 1.000000000000000000, 0.000000000000000000, 0.000000000000000000 ) ) ;
#9874=ORIENTED_EDGE ( 'NONE', *, *, #8625, .F. ) ;
#9894=DIRECTION ( 'NONE',  ( 1.000000000000000000, 0.000000000000000000, 0.000000000000000000 ) ) ;
#9895=FILL_AREA_STYLE ('',( #13477 ) ) ;
#9942=FACE_BOUND ( 'NONE', #10070, .T. ) ;
#9954=VECTOR ( 'NONE', #455, 1000.000000000000000 ) ;
#9959=LINE ( 'NONE', #4287, #10721 ) ;
#9998=AXIS2_PLACEMENT_3D ( 'NONE', #1555, #3688, #11968 ) ;
#10015=UNCERTAINTY_MEASURE_WITH_UNIT (LENGTH_MEASURE( 1.000000000000000082E-05 ), #7698, 'distance_accuracy_value', 'NONE');
#10037=VECTOR ( 'NONE', #1329, 1000.000000000000000 ) ;
#10065=ORIENTED_EDGE ( 'NONE', *, *, #11192, .F. ) ;
#10070=EDGE_LOOP ( 'NONE', ( #4307, #1779 ) ) ;
#10110=EDGE_CURVE ( 'NONE', #1622, #1196, #2675, .T. ) ;
#10117=VERTEX_POINT ( 'NONE', #13142 ) ;
#10146=FACE_OUTER_BOUND ( 'NONE', #10633, .T. ) ;
#10187=ORIENTED_EDGE ( 'NONE', *, *, #6012, .T. ) ;
#10219=ORIENTED_EDGE ( 'NONE', *, *, #5242, .F. ) ;
#10225=FILL_AREA_STYLE_COLOUR ( '', #11142 ) ;
#10254=CARTESIAN_POINT ( 'NONE',  ( -20.00000000000000000, 2.449293598294706513E-15, -43.49999999999998579 ) ) ;
#10403=AXIS2_PLACEMENT_3D ( 'NONE', #14435, #8501, #2883 ) ;
#10409=CARTESIAN_POINT ( 'NONE',  ( -22.33583958711380646, -30.74264578624812927, -25.50000000000000355 ) ) ;
#10426=DIRECTION ( 'NONE',  ( -0.000000000000000000, -0.000000000000000000, -1.000000000000000000 ) ) ;
#10448=SURFACE_SIDE_STYLE ('',( #6793 ) ) ;
#10473=VECTOR ( 'NONE', #9324, 1000.000000000000000 ) ;
#10509=CIRCLE ( 'NONE', #2269, 2.649999999999985700 ) ;
#10520=CARTESIAN_POINT ( 'NONE',  ( -36.14014761921588104, 11.74264578624790190, -25.50000000000000355 ) ) ;
#10596=EDGE_CURVE ( 'NONE', #13414, #5762, #2689, .T. ) ;
#10604=VERTEX_POINT ( 'NONE', #11997 ) ;
#10633=EDGE_LOOP ( 'NONE', ( #6716, #2463, #1850, #1443 ) ) ;
#10643=CARTESIAN_POINT ( 'NONE',  ( -14.00000000000000000, 0.000000000000000000, 14.49999999999999822 ) ) ;
#10657=AXIS2_PLACEMENT_3D ( 'NONE', #10409, #13841, #4575 ) ;
#10721=VECTOR ( 'NONE', #4208, 1000.000000000000000 ) ;
#10726=DIRECTION ( 'NONE',  ( 0.000000000000000000, 0.000000000000000000, 1.000000000000000000 ) ) ;
#10728=CARTESIAN_POINT ( 'NONE',  ( 0.000000000000000000, 0.000000000000000000, -45.50000000000000000 ) ) ;
#10732=CARTESIAN_POINT ( 'NONE',  ( 0.000000000000000000, 0.000000000000000000, -45.50000000000000000 ) ) ;
#10743=VERTEX_POINT ( 'NONE', #11222 ) ;
#10752=VERTEX_POINT ( 'NONE', #1806 ) ;
#10768=DIRECTION ( 'NONE',  ( 1.000000000000000000, 0.000000000000000000, 0.000000000000000000 ) ) ;
#10769=ORIENTED_EDGE ( 'NONE', *, *, #722, .F. ) ;
#10778=CARTESIAN_POINT ( 'NONE',  ( 0.000000000000000000, 0.000000000000000000, -45.50000000000000000 ) ) ;
#10824=FACE_OUTER_BOUND ( 'NONE', #13316, .T. ) ;
#10869=ORIENTED_EDGE ( 'NONE', *, *, #9617, .T. ) ;
#10892=FACE_BOUND ( 'NONE', #11278, .T. ) ;
#10920=ORIENTED_EDGE ( 'NONE', *, *, #12563, .T. ) ;
#10968=DIRECTION ( 'NONE',  ( -0.000000000000000000, -0.000000000000000000, -1.000000000000000000 ) ) ;
#10970=AXIS2_PLACEMENT_3D ( 'NONE', #3977, #1691, #3905 ) ;
#10972=DIRECTION ( 'NONE',  ( -0.000000000000000000, -0.000000000000000000, -1.000000000000000000 ) ) ;
#10978=AXIS2_PLACEMENT_3D ( 'NONE', #4248, #11145, #5526 ) ;
#11006=CIRCLE ( 'NONE', #4472, 44.89637028918153305 ) ;
#11074=LINE ( 'NONE', #5296, #13643 ) ;
#11088=PRODUCT_DEFINITION_CONTEXT ( 'detailed design', #5236, 'design' ) ;
#11099=ORIENTED_EDGE ( 'NONE', *, *, #11826, .F. ) ;
#11127=ADVANCED_FACE ( 'NONE', ( #12837 ), #4871, .F. ) ;
#11142=COLOUR_RGB ( '', 0.08235294, 0.09019608, 0.10196078) ;
#11145=DIRECTION ( 'NONE',  ( -0.000000000000000000, -0.000000000000000000, 1.000000000000000000 ) ) ;
#11158=CIRCLE ( 'NONE', #7015, 20.00000000000000000 ) ;
#11180=EDGE_CURVE ( 'NONE', #4586, #2764, #9268, .T. ) ;
#11187=CARTESIAN_POINT ( 'NONE',  ( -36.14014761921588104, 11.74264578624790190, 14.49999999999999822 ) ) ;
#11192=EDGE_CURVE ( 'NONE', #7885, #5519, #14130, .T. ) ;
#11222=CARTESIAN_POINT ( 'NONE',  ( -33.49014761921589667, 11.74264578624790190, -25.50000000000000355 ) ) ;
#11242=CARTESIAN_POINT ( 'NONE',  ( 0.000000000000000000, 0.000000000000000000, -45.50000000000000000 ) ) ;
#11262=AXIS2_PLACEMENT_3D ( 'NONE', #1877, #2030, #2106 ) ;
#11273=AXIS2_PLACEMENT_3D ( 'NONE', #5676, #13739, #9239 ) ;
#11278=EDGE_LOOP ( 'NONE', ( #12803, #357 ) ) ;
#11293=CARTESIAN_POINT ( 'NONE',  ( -19.68583958711381854, -30.74264578624812927, 14.49999999999999822 ) ) ;
#11304=CYLINDRICAL_SURFACE ( 'NONE', #10978, 20.00000000000000000 ) ;
#11349=CARTESIAN_POINT ( 'NONE',  ( 38.79014761921568777, 11.74264578624841171, 14.49999999999999822 ) ) ;
#11407=VECTOR ( 'NONE', #3033, 1000.000000000000000 ) ;
#11438=EDGE_LOOP ( 'NONE', ( #12527, #7083, #14862, #10065 ) ) ;
#11456=ADVANCED_FACE ( 'NONE', ( #6506 ), #2553, .T. ) ;
#11466=VERTEX_POINT ( 'NONE', #3265 ) ;
#11521=ORIENTED_EDGE ( 'NONE', *, *, #1846, .F. ) ;
#11542=DIRECTION ( 'NONE',  ( -1.000000000000000000, 0.000000000000000000, 0.000000000000000000 ) ) ;
#11600=EDGE_CURVE ( 'NONE', #10752, #10743, #2345, .T. ) ;
#11613=ORIENTED_EDGE ( 'NONE', *, *, #722, .T. ) ;
#11615=CARTESIAN_POINT ( 'NONE',  ( 14.00000000000000000, 1.714505518806294638E-15, 14.49999999999999822 ) ) ;
#11617=VERTEX_POINT ( 'NONE', #2492 ) ;
#11618=EDGE_LOOP ( 'NONE', ( #9177, #7596, #8516, #10219 ) ) ;
#11630=AXIS2_PLACEMENT_3D ( 'NONE', #8362, #2741, #12018 ) ;
#11684=EDGE_CURVE ( 'NONE', #13374, #11825, #6045, .T. ) ;
#11696=DIRECTION ( 'NONE',  ( -1.000000000000000000, 0.000000000000000000, 0.000000000000000000 ) ) ;
#11699=VERTEX_POINT ( 'NONE', #6201 ) ;
#11702=AXIS2_PLACEMENT_3D ( 'NONE', #2491, #10972, #11696 ) ;
#11754=CONICAL_SURFACE ( 'NONE', #11273, 18.00000000000000355, 0.7853981633974439491 ) ;
#11773=CIRCLE ( 'NONE', #615, 14.00000000000000000 ) ;
#11774=DIRECTION ( 'NONE',  ( 1.000000000000000000, 0.000000000000000000, 0.000000000000000000 ) ) ;
#11796=ORIENTED_EDGE ( 'NONE', *, *, #1832, .F. ) ;
#11819=EDGE_LOOP ( 'NONE', ( #5982, #3484, #2954, #12530 ) ) ;
#11825=VERTEX_POINT ( 'NONE', #4394 ) ;
#11826=EDGE_CURVE ( 'NONE', #5585, #9114, #2770, .T. ) ;
#11839=CARTESIAN_POINT ( 'NONE',  ( 0.000000000000000000, 0.000000000000000000, -45.50000000000000000 ) ) ;
#11872=MECHANICAL_DESIGN_GEOMETRIC_PRESENTATION_REPRESENTATION('',(#2405),#15026);
#11919=DIRECTION ( 'NONE',  ( -1.000000000000000000, 0.000000000000000000, 0.000000000000000000 ) ) ;
#11932=DIRECTION ( 'NONE',  ( -1.000000000000000000, 0.000000000000000000, 0.000000000000000000 ) ) ;
#11962=LINE ( 'NONE', #6167, #10037 ) ;
#11963=EDGE_CURVE ( 'NONE', #6056, #7966, #7820, .T. ) ;
#11968=DIRECTION ( 'NONE',  ( -1.000000000000000000, 0.000000000000000000, 0.000000000000000000 ) ) ;
#11997=CARTESIAN_POINT ( 'NONE',  ( 2.649999999999987033, 38.00000000000000000, -25.50000000000000355 ) ) ;
#12018=DIRECTION ( 'NONE',  ( 1.000000000000000000, 0.000000000000000000, 0.000000000000000000 ) ) ;
#12057=CYLINDRICAL_SURFACE ( 'NONE', #7629, 2.649999999999985700 ) ;
#12076=EDGE_LOOP ( 'NONE', ( #11796, #551, #8442, #12642 ) ) ;
#12084=CARTESIAN_POINT ( 'NONE',  ( -24.98583958711379083, -30.74264578624812927, 14.49999999999999822 ) ) ;
#12100=ADVANCED_FACE ( 'NONE', ( #10892, #496, #3779, #8397, #6025, #8461, #10824 ), #9662, .F. ) ;
#12119=LINE ( 'NONE', #7172, #7153 ) ;
#12272=ORIENTED_EDGE ( 'NONE', *, *, #4676, .F. ) ;
#12274=SURFACE_STYLE_FILL_AREA ( #9895 ) ;
#12314=DIRECTION ( 'NONE',  ( -1.000000000000000000, 0.000000000000000000, 0.000000000000000000 ) ) ;
#12319=ORIENTED_EDGE ( 'NONE', *, *, #12870, .F. ) ;
#12322=ORIENTED_EDGE ( 'NONE', *, *, #12870, .T. ) ;
#12347=EDGE_CURVE ( 'NONE', #10604, #10117, #3493, .T. ) ;
#12454=AXIS2_PLACEMENT_3D ( 'NONE', #10732, #255, #3907 ) ;
#12500=ORIENTED_EDGE ( 'NONE', *, *, #12526, .F. ) ;
#12526=EDGE_CURVE ( 'NONE', #1196, #1622, #6623, .T. ) ;
#12527=ORIENTED_EDGE ( 'NONE', *, *, #7924, .T. ) ;
#12530=ORIENTED_EDGE ( 'NONE', *, *, #1022, .F. ) ;
#12538=FACE_BOUND ( 'NONE', #9688, .T. ) ;
#12563=EDGE_CURVE ( 'NONE', #1453, #11466, #2276, .T. ) ;
#12601=DIRECTION ( 'NONE',  ( -0.000000000000000000, -0.000000000000000000, -1.000000000000000000 ) ) ;
#12602=VERTEX_POINT ( 'NONE', #1551 ) ;
#12642=ORIENTED_EDGE ( 'NONE', *, *, #8604, .T. ) ;
#12665=EDGE_CURVE ( 'NONE', #1453, #5585, #11962, .T. ) ;
#12674=DIRECTION ( 'NONE',  ( 1.000000000000000000, 0.000000000000000000, 0.000000000000000000 ) ) ;
#12681=DIRECTION ( 'NONE',  ( -0.000000000000000000, -0.000000000000000000, -1.000000000000000000 ) ) ;
#12737=VECTOR ( 'NONE', #3511, 1000.000000000000000 ) ;
#12740=FILL_AREA_STYLE ('',( #10225 ) ) ;
#12803=ORIENTED_EDGE ( 'NONE', *, *, #2861, .F. ) ;
#12811=DIRECTION ( 'NONE',  ( -0.000000000000000000, -0.000000000000000000, -1.000000000000000000 ) ) ;
#12837=FACE_OUTER_BOUND ( 'NONE', #6158, .T. ) ;
#12870=EDGE_CURVE ( 'NONE', #4586, #664, #584, .T. ) ;
#12873=ORIENTED_EDGE ( 'NONE', *, *, #12665, .T. ) ;
#12889=LINE ( 'NONE', #1140, #4804 ) ;
#12904=DIRECTION ( 'NONE',  ( 0.000000000000000000, 0.000000000000000000, 1.000000000000000000 ) ) ;
#12927=DIRECTION ( 'NONE',  ( -0.000000000000000000, -0.000000000000000000, -1.000000000000000000 ) ) ;
#12931=AXIS2_PLACEMENT_3D ( 'NONE', #2204, #6820, #8950 ) ;
#12937=VERTEX_POINT ( 'NONE', #3290 ) ;
#12943=CARTESIAN_POINT ( 'NONE',  ( 0.000000000000000000, 0.000000000000000000, -43.49999999999998579 ) ) ;
#12944=ORIENTED_EDGE ( 'NONE', *, *, #6310, .T. ) ;
#12972=AXIS2_PLACEMENT_3D ( 'NONE', #5044, #13024, #14236 ) ;
#12990=ORIENTED_EDGE ( 'NONE', *, *, #8625, .T. ) ;
#12991=ORIENTED_EDGE ( 'NONE', *, *, #6230, .T. ) ;
#13005=AXIS2_PLACEMENT_3D ( 'NONE', #5580, #9148, #1181 ) ;
#13024=DIRECTION ( 'NONE',  ( 0.000000000000000000, 0.000000000000000000, -1.000000000000000000 ) ) ;
#13058=VERTEX_POINT ( 'NONE', #9686 ) ;
#13074=ORIENTED_EDGE ( 'NONE', *, *, #792, .F. ) ;
#13142=CARTESIAN_POINT ( 'NONE',  ( -2.649999999999987921, 38.00000000000000000, -25.50000000000000355 ) ) ;
#13146=CYLINDRICAL_SURFACE ( 'NONE', #5095, 14.00000000000000000 ) ;
#13165=AXIS2_PLACEMENT_3D ( 'NONE', #11187, #786, #7750 ) ;
#13241=DIRECTION ( 'NONE',  ( -1.000000000000000000, 0.000000000000000000, -0.000000000000000000 ) ) ;
#13249=UNCERTAINTY_MEASURE_WITH_UNIT (LENGTH_MEASURE( 1.000000000000000082E-05 ), #908, 'distance_accuracy_value', 'NONE');
#13263=DIRECTION ( 'NONE',  ( 1.000000000000000000, 0.000000000000000000, 0.000000000000000000 ) ) ;
#13290=ADVANCED_FACE ( 'NONE', ( #14386 ), #8534, .F. ) ;
#13316=EDGE_LOOP ( 'NONE', ( #14109, #9673 ) ) ;
#13350=EDGE_CURVE ( 'NONE', #13058, #6851, #2459, .T. ) ;
#13374=VERTEX_POINT ( 'NONE', #11349 ) ;
#13383=AXIS2_PLACEMENT_3D ( 'NONE', #3358, #943, #4435 ) ;
#13414=VERTEX_POINT ( 'NONE', #13474 ) ;
#13448=CARTESIAN_POINT ( 'NONE',  ( 0.000000000000000000, 0.000000000000000000, 14.49999999999999822 ) ) ;
#13470=AXIS2_PLACEMENT_3D ( 'NONE', #11242, #4488, #6667 ) ;
#13474=CARTESIAN_POINT ( 'NONE',  ( 14.00000000000000000, 1.714505518806294638E-15, -45.50000000000000000 ) ) ;
#13477=FILL_AREA_STYLE_COLOUR ( '', #7307 ) ;
#13521=DIRECTION ( 'NONE',  ( 1.000000000000000000, 0.000000000000000000, 0.000000000000000000 ) ) ;
#13564=AXIS2_PLACEMENT_3D ( 'NONE', #6816, #12601, #13904 ) ;
#13571=DIRECTION ( 'NONE',  ( 0.000000000000000000, 0.000000000000000000, 1.000000000000000000 ) ) ;
#13639=MECHANICAL_DESIGN_GEOMETRIC_PRESENTATION_REPRESENTATION('',(#796),#2241);
#13643=VECTOR ( 'NONE', #4173, 1000.000000000000000 ) ;
#13644=AXIS2_PLACEMENT_3D ( 'NONE', #9714, #3670, #7216 ) ;
#13648=( NAMED_UNIT ( * ) SI_UNIT ( $, .STERADIAN. ) SOLID_ANGLE_UNIT ( ) );
#13678=ORIENTED_EDGE ( 'NONE', *, *, #13873, .F. ) ;
#13738=ORIENTED_EDGE ( 'NONE', *, *, #11192, .T. ) ;
#13739=DIRECTION ( 'NONE',  ( 0.000000000000000000, 0.000000000000000000, 1.000000000000000000 ) ) ;
#13812=ORIENTED_EDGE ( 'NONE', *, *, #12526, .T. ) ;
#13813=CARTESIAN_POINT ( 'NONE',  ( 24.98583958711423492, -30.74264578624780597, 14.49999999999999822 ) ) ;
#13841=DIRECTION ( 'NONE',  ( -0.000000000000000000, -0.000000000000000000, -1.000000000000000000 ) ) ;
#13859=CARTESIAN_POINT ( 'NONE',  ( 22.33583958711425055, -30.74264578624780597, -25.50000000000000355 ) ) ;
#13873=EDGE_CURVE ( 'NONE', #12602, #5519, #289, .T. ) ;
#13875=EDGE_CURVE ( 'NONE', #5875, #7688, #5205, .T. ) ;
#13897=EDGE_LOOP ( 'NONE', ( #2209, #1989, #6252, #9129 ) ) ;
#13904=DIRECTION ( 'NONE',  ( -1.000000000000000000, 0.000000000000000000, 0.000000000000000000 ) ) ;
#13924=SHAPE_DEFINITION_REPRESENTATION ( #7533, #1232 ) ;
#13958=DIRECTION ( 'NONE',  ( -0.000000000000000000, -0.000000000000000000, -1.000000000000000000 ) ) ;
#14003=ORIENTED_EDGE ( 'NONE', *, *, #6210, .T. ) ;
#14006=MANIFOLD_SOLID_BREP ( 'M5 Clearance Hole1', #434 ) ;
#14019=ORIENTED_EDGE ( 'NONE', *, *, #14320, .F. ) ;
#14041=ORIENTED_EDGE ( 'NONE', *, *, #2993, .F. ) ;
#14044=ORIENTED_EDGE ( 'NONE', *, *, #7073, .F. ) ;
#14109=ORIENTED_EDGE ( 'NONE', *, *, #5367, .F. ) ;
#14130=LINE ( 'NONE', #1304, #6174 ) ;
#14162=ORIENTED_EDGE ( 'NONE', *, *, #4327, .T. ) ;
#14180=ADVANCED_FACE ( 'NONE', ( #7379 ), #7300, .F. ) ;
#14213=DIRECTION ( 'NONE',  ( -1.000000000000000000, 0.000000000000000000, 0.000000000000000000 ) ) ;
#14236=DIRECTION ( 'NONE',  ( -1.000000000000000000, 0.000000000000000000, 0.000000000000000000 ) ) ;
#14253=DIRECTION ( 'NONE',  ( 1.000000000000000000, 0.000000000000000000, 0.000000000000000000 ) ) ;
#14261=DIRECTION ( 'NONE',  ( -0.000000000000000000, -0.000000000000000000, -1.000000000000000000 ) ) ;
#14276=CARTESIAN_POINT ( 'NONE',  ( 18.00000000000000355, 0.000000000000000000, -45.50000000000000000 ) ) ;
#14277=CARTESIAN_POINT ( 'NONE',  ( 0.000000000000000000, 0.000000000000000000, 14.49999999999999822 ) ) ;
#14284=FACE_OUTER_BOUND ( 'NONE', #5481, .T. ) ;
#14312=DIRECTION ( 'NONE',  ( 0.000000000000000000, 0.000000000000000000, 1.000000000000000000 ) ) ;
#14318=FACE_OUTER_BOUND ( 'NONE', #5006, .T. ) ;
#14320=EDGE_CURVE ( 'NONE', #11466, #9114, #9959, .T. ) ;
#14359=EDGE_CURVE ( 'NONE', #10752, #5875, #2727, .T. ) ;
#14386=FACE_OUTER_BOUND ( 'NONE', #13897, .T. ) ;
#14398=DIRECTION ( 'NONE',  ( -1.000000000000000000, 0.000000000000000000, 0.000000000000000000 ) ) ;
#14435=CARTESIAN_POINT ( 'NONE',  ( -22.33583958711380646, -30.74264578624812927, 14.49999999999999822 ) ) ;
#14452=VECTOR ( 'NONE', #141, 1000.000000000000000 ) ;
#14480=DIRECTION ( 'NONE',  ( 0.000000000000000000, 0.000000000000000000, 1.000000000000000000 ) ) ;
#14509=ADVANCED_FACE ( 'NONE', ( #3286 ), #7054, .F. ) ;
#14515=DIRECTION ( 'NONE',  ( 0.000000000000000000, 0.000000000000000000, 1.000000000000000000 ) ) ;
#14557=ADVANCED_FACE ( 'NONE', ( #7207 ), #391, .F. ) ;
#14593=FACE_BOUND ( 'NONE', #2191, .T. ) ;
#14596=CARTESIAN_POINT ( 'NONE',  ( 36.14014761921570340, 11.74264578624841171, -25.50000000000000355 ) ) ;
#14641=CIRCLE ( 'NONE', #12931, 2.649999999999985700 ) ;
#14665=ADVANCED_FACE ( 'NONE', ( #1386 ), #13146, .F. ) ;
#14730=VERTEX_POINT ( 'NONE', #1824 ) ;
#14788=SURFACE_STYLE_USAGE ( .BOTH. , #10448 ) ;
#14862=ORIENTED_EDGE ( 'NONE', *, *, #13873, .T. ) ;
#14868=DIRECTION ( 'NONE',  ( -0.000000000000000000, -0.000000000000000000, -1.000000000000000000 ) ) ;
#14870=CARTESIAN_POINT ( 'NONE',  ( -36.14014761921588104, 11.74264578624790190, -25.50000000000000355 ) ) ;
#14885=AXIS2_PLACEMENT_3D ( 'NONE', #2926, #1793, #6401 ) ;
#14918=CIRCLE ( 'NONE', #12972, 20.00000000000000000 ) ;
#14926=( NAMED_UNIT ( * ) PLANE_ANGLE_UNIT ( ) SI_UNIT ( $, .RADIAN. ) );
#15014=CARTESIAN_POINT ( 'NONE',  ( -2.449293598294708880E-16, 38.00000000000000000, 14.49999999999999822 ) ) ;
#15026=( GEOMETRIC_REPRESENTATION_CONTEXT ( 3 ) GLOBAL_UNCERTAINTY_ASSIGNED_CONTEXT ( ( #1700 ) ) GLOBAL_UNIT_ASSIGNED_CONTEXT ( ( #4612, #9157, #13648 ) ) REPRESENTATION_CONTEXT ( 'NONE', 'WORKASPACE' ) );
#15028=EDGE_LOOP ( 'NONE', ( #6398, #8836 ) ) ;
ENDSEC;
END-ISO-10303-21;
